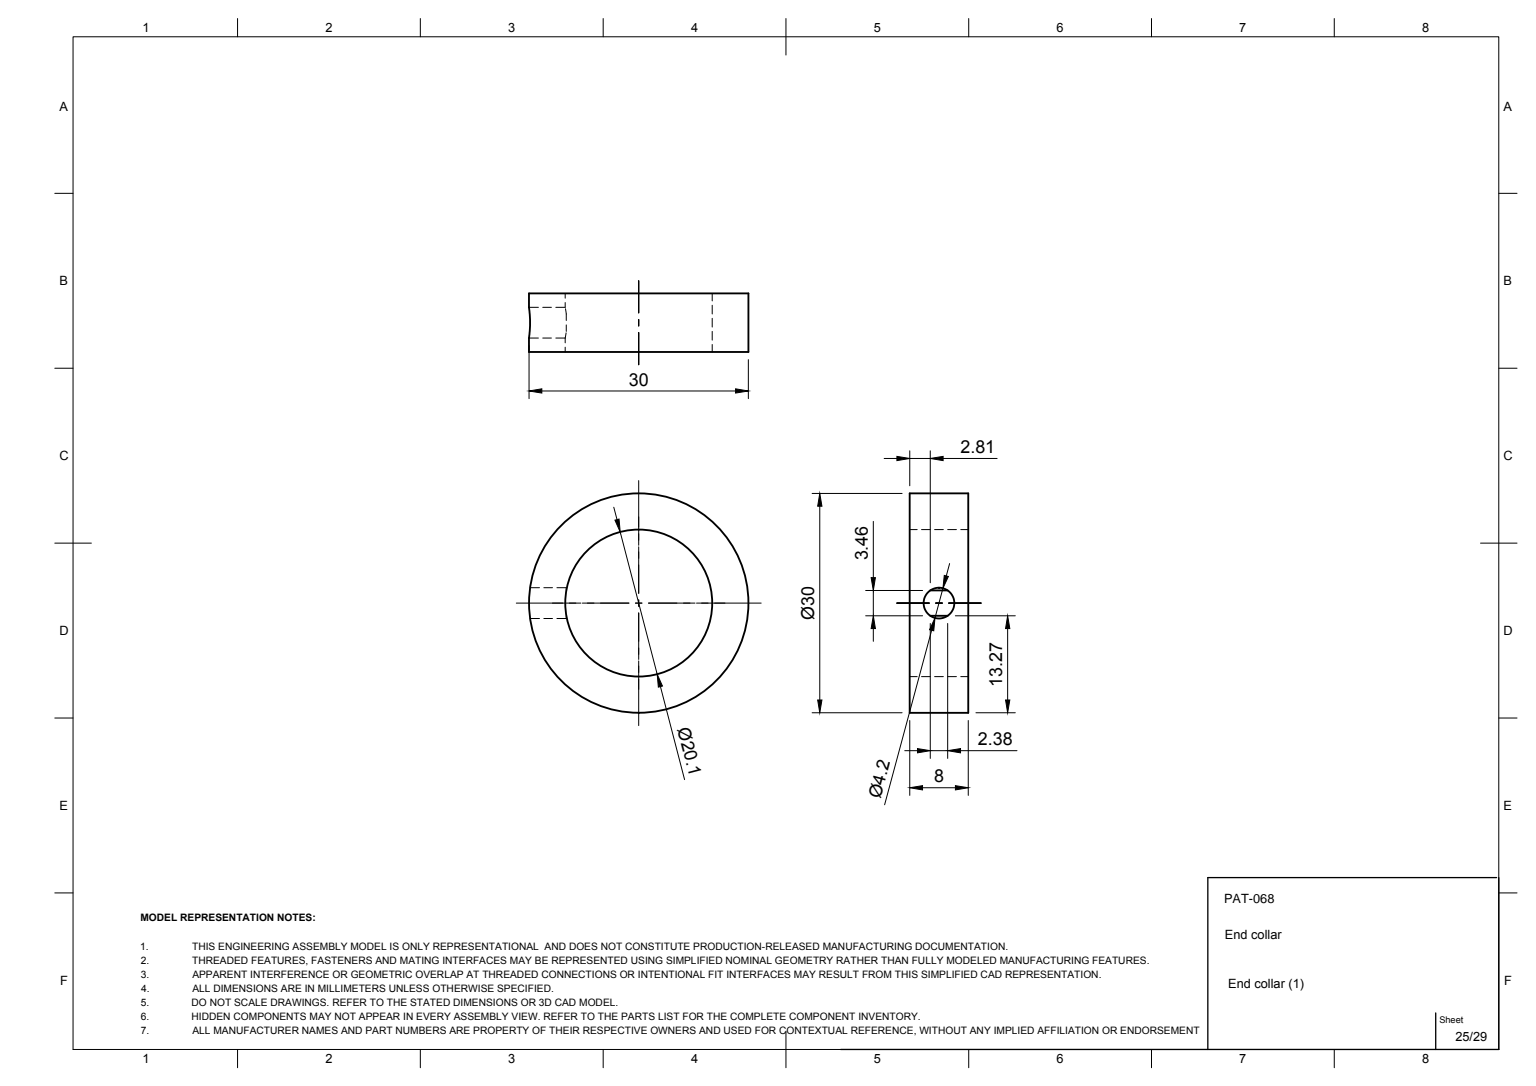
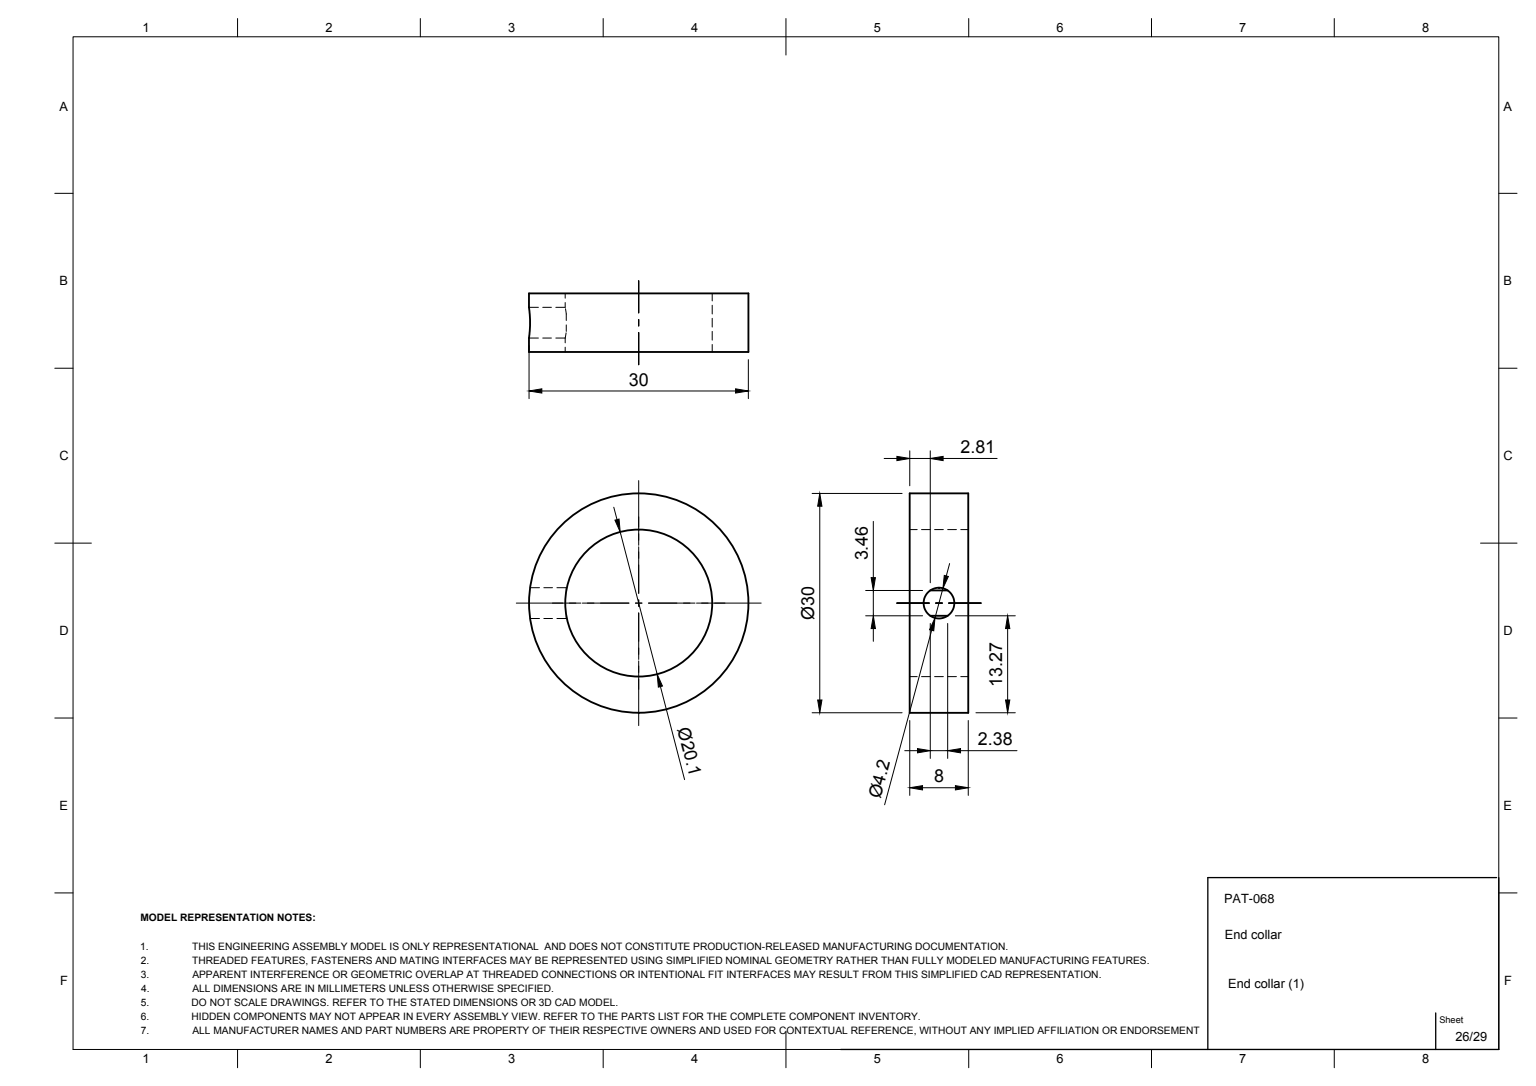
ISO-10303-21;
HEADER;
/* Generated by software containing ST-Developer
 * from STEP Tools, Inc. (www.steptools.com) 
 */

FILE_DESCRIPTION(
/* description */ ('Line shaft on three pillow blocks'),
/* implementation_level */ '2;1');

FILE_NAME(
/* name */ 'End collar.step',
/* time_stamp */ '2026-10-27T10:49:19-07:00',
/* author */ (''),
/* organization */ (''),
/* preprocessor_version */ 'ST-DEVELOPER v20.2',
/* originating_system */ 'Autodesk Translation Framework v15.17.0.0',
/* authorisation */ '');

FILE_SCHEMA (('AUTOMOTIVE_DESIGN { 1 0 10303 214 3 1 1 }'));
ENDSEC;

DATA;
#10=MECHANICAL_DESIGN_GEOMETRIC_PRESENTATION_REPRESENTATION('',(#359),#8377);
#255=B_SPLINE_CURVE_WITH_KNOTS('',3,(#7910,#7911,#7912,#7913,#7914,#7915,
#7916,#7917,#7918,#7919,#7920,#7921,#7922,#7923),.UNSPECIFIED.,.F.,.F.,
(4,2,2,2,2,2,4),(0.75600573798702,0.793568827564647,0.872922520054201,0.952276212543756,
1.03162990503331,1.11098359752287,1.14854668710049),.UNSPECIFIED.);
#256=B_SPLINE_CURVE_WITH_KNOTS('',3,(#7929,#7930,#7931,#7932,#7933,#7934,
#7935,#7936,#7937,#7938,#7939,#7940,#7941,#7942,#7943,#7944,#7945,#7946),
 .UNSPECIFIED.,.F.,.F.,(4,2,2,2,2,2,2,2,4),(0.,0.079216580773363,0.158433161546726,
0.23764869707457,0.316864232602414,0.396079768130259,0.475295303658103,
0.554511884431466,0.633728465204829),.UNSPECIFIED.);
#257=B_SPLINE_CURVE_WITH_KNOTS('',3,(#7947,#7948,#7949,#7950,#7951,#7952,
#7953,#7954,#7955,#7956,#7957,#7958,#7959,#7960,#7961,#7962,#7963,#7964),
 .UNSPECIFIED.,.F.,.F.,(4,2,2,2,2,2,2,2,4),(0.633728465204829,0.712945045978192,
0.792161626751555,0.871377162279399,0.950592697807244,1.02980823333509,
1.10902376886293,1.18824034963629,1.26745693040966),.UNSPECIFIED.);
#258=B_SPLINE_CURVE_WITH_KNOTS('',3,(#7967,#7968,#7969,#7970,#7971,#7972,
#7973,#7974,#7975,#7976,#7977,#7978,#7979,#7980),.UNSPECIFIED.,.F.,.F.,
(4,2,2,2,2,2,4),(0.121154929624515,0.158718019202143,0.238071711691697,
0.317425404181252,0.396779096670807,0.476132789160362,0.513695878737989),
 .UNSPECIFIED.);
#304=SHAPE_REPRESENTATION_RELATIONSHIP('SRR','None',#8521,#331);
#331=ADVANCED_BREP_SHAPE_REPRESENTATION('',(#385),#8370);
#359=STYLED_ITEM('',(#8704),#385);
#385=MANIFOLD_SOLID_BREP('Body1',#4347);
#474=FACE_BOUND('',#1184,.T.);
#475=FACE_BOUND('',#1186,.T.);
#476=FACE_BOUND('',#1188,.T.);
#477=FACE_BOUND('',#1190,.T.);
#612=PLANE('',#5030);
#613=PLANE('',#5035);
#614=PLANE('',#5042);
#615=PLANE('',#5043);
#845=FACE_OUTER_BOUND('',#1180,.T.);
#846=FACE_OUTER_BOUND('',#1181,.T.);
#847=FACE_OUTER_BOUND('',#1182,.T.);
#848=FACE_OUTER_BOUND('',#1183,.T.);
#849=FACE_OUTER_BOUND('',#1185,.T.);
#850=FACE_OUTER_BOUND('',#1187,.T.);
#851=FACE_OUTER_BOUND('',#1189,.T.);
#1180=EDGE_LOOP('',(#3751,#3752));
#1181=EDGE_LOOP('',(#3753,#3754,#3755,#3756,#3757,#3758,#3759,#3760,#3761));
#1182=EDGE_LOOP('',(#3762,#3763,#3764));
#1183=EDGE_LOOP('',(#3765,#3766,#3767,#3768));
#1184=EDGE_LOOP('',(#3769,#3770,#3771,#3772));
#1185=EDGE_LOOP('',(#3773,#3774,#3775,#3776));
#1186=EDGE_LOOP('',(#3777,#3778));
#1187=EDGE_LOOP('',(#3779));
#1188=EDGE_LOOP('',(#3780));
#1189=EDGE_LOOP('',(#3781));
#1190=EDGE_LOOP('',(#3782));
#1499=LINE('',#7906,#1826);
#1500=LINE('',#7927,#1827);
#1501=LINE('',#7982,#1828);
#1502=LINE('',#7987,#1829);
#1503=LINE('',#7993,#1830);
#1826=VECTOR('',#6148,1.);
#1827=VECTOR('',#6155,0.21);
#1828=VECTOR('',#6160,1.);
#1829=VECTOR('',#6165,1.005);
#1830=VECTOR('',#6172,1.5);
#2034=CIRCLE('',#5031,0.21);
#2035=CIRCLE('',#5033,0.21);
#2036=CIRCLE('',#5034,0.21);
#2037=CIRCLE('',#5037,1.005);
#2038=CIRCLE('',#5038,1.005);
#2039=CIRCLE('',#5040,1.5);
#2040=CIRCLE('',#5041,1.5);
#2341=VERTEX_POINT('',#7904);
#2342=VERTEX_POINT('',#7905);
#2343=VERTEX_POINT('',#7909);
#2344=VERTEX_POINT('',#7924);
#2345=VERTEX_POINT('',#7926);
#2346=VERTEX_POINT('',#7928);
#2347=VERTEX_POINT('',#7965);
#2348=VERTEX_POINT('',#7984);
#2349=VERTEX_POINT('',#7986);
#2350=VERTEX_POINT('',#7990);
#2351=VERTEX_POINT('',#7992);
#2824=EDGE_CURVE('',#2341,#2342,#1499,.T.);
#2825=EDGE_CURVE('',#2341,#2342,#2034,.T.);
#2826=EDGE_CURVE('',#2343,#2341,#255,.T.);
#2827=EDGE_CURVE('',#2344,#2343,#2035,.T.);
#2828=EDGE_CURVE('',#2344,#2345,#1500,.T.);
#2829=EDGE_CURVE('',#2346,#2345,#256,.T.);
#2830=EDGE_CURVE('',#2345,#2346,#257,.T.);
#2831=EDGE_CURVE('',#2347,#2344,#2036,.T.);
#2832=EDGE_CURVE('',#2342,#2347,#258,.T.);
#2833=EDGE_CURVE('',#2347,#2343,#1501,.T.);
#2834=EDGE_CURVE('',#2348,#2348,#2037,.T.);
#2835=EDGE_CURVE('',#2348,#2349,#1502,.T.);
#2836=EDGE_CURVE('',#2349,#2349,#2038,.T.);
#2837=EDGE_CURVE('',#2350,#2350,#2039,.T.);
#2838=EDGE_CURVE('',#2350,#2351,#1503,.T.);
#2839=EDGE_CURVE('',#2351,#2351,#2040,.T.);
#3751=ORIENTED_EDGE('',*,*,#2824,.F.);
#3752=ORIENTED_EDGE('',*,*,#2825,.T.);
#3753=ORIENTED_EDGE('',*,*,#2826,.F.);
#3754=ORIENTED_EDGE('',*,*,#2827,.F.);
#3755=ORIENTED_EDGE('',*,*,#2828,.T.);
#3756=ORIENTED_EDGE('',*,*,#2829,.F.);
#3757=ORIENTED_EDGE('',*,*,#2830,.F.);
#3758=ORIENTED_EDGE('',*,*,#2828,.F.);
#3759=ORIENTED_EDGE('',*,*,#2831,.F.);
#3760=ORIENTED_EDGE('',*,*,#2832,.F.);
#3761=ORIENTED_EDGE('',*,*,#2825,.F.);
#3762=ORIENTED_EDGE('',*,*,#2833,.F.);
#3763=ORIENTED_EDGE('',*,*,#2831,.T.);
#3764=ORIENTED_EDGE('',*,*,#2827,.T.);
#3765=ORIENTED_EDGE('',*,*,#2834,.F.);
#3766=ORIENTED_EDGE('',*,*,#2835,.T.);
#3767=ORIENTED_EDGE('',*,*,#2836,.T.);
#3768=ORIENTED_EDGE('',*,*,#2835,.F.);
#3769=ORIENTED_EDGE('',*,*,#2832,.T.);
#3770=ORIENTED_EDGE('',*,*,#2833,.T.);
#3771=ORIENTED_EDGE('',*,*,#2826,.T.);
#3772=ORIENTED_EDGE('',*,*,#2824,.T.);
#3773=ORIENTED_EDGE('',*,*,#2837,.F.);
#3774=ORIENTED_EDGE('',*,*,#2838,.T.);
#3775=ORIENTED_EDGE('',*,*,#2839,.T.);
#3776=ORIENTED_EDGE('',*,*,#2838,.F.);
#3777=ORIENTED_EDGE('',*,*,#2829,.T.);
#3778=ORIENTED_EDGE('',*,*,#2830,.T.);
#3779=ORIENTED_EDGE('',*,*,#2837,.T.);
#3780=ORIENTED_EDGE('',*,*,#2834,.T.);
#3781=ORIENTED_EDGE('',*,*,#2839,.F.);
#3782=ORIENTED_EDGE('',*,*,#2836,.F.);
#4059=CYLINDRICAL_SURFACE('',#5032,0.21);
#4060=CYLINDRICAL_SURFACE('',#5036,1.005);
#4061=CYLINDRICAL_SURFACE('',#5039,1.5);
#4263=ADVANCED_FACE('',(#845),#612,.T.);
#4264=ADVANCED_FACE('',(#846),#4059,.F.);
#4265=ADVANCED_FACE('',(#847),#613,.T.);
#4266=ADVANCED_FACE('',(#848,#474),#4060,.F.);
#4267=ADVANCED_FACE('',(#849,#475),#4061,.T.);
#4268=ADVANCED_FACE('',(#850,#476),#614,.T.);
#4269=ADVANCED_FACE('',(#851,#477),#615,.F.);
#4347=CLOSED_SHELL('',(#4263,#4264,#4265,#4266,#4267,#4268,#4269));
#5029=AXIS2_PLACEMENT_3D('',#7902,#6144,#6145);
#5030=AXIS2_PLACEMENT_3D('',#7903,#6146,#6147);
#5031=AXIS2_PLACEMENT_3D('',#7907,#6149,#6150);
#5032=AXIS2_PLACEMENT_3D('',#7908,#6151,#6152);
#5033=AXIS2_PLACEMENT_3D('',#7925,#6153,#6154);
#5034=AXIS2_PLACEMENT_3D('',#7966,#6156,#6157);
#5035=AXIS2_PLACEMENT_3D('',#7981,#6158,#6159);
#5036=AXIS2_PLACEMENT_3D('',#7983,#6161,#6162);
#5037=AXIS2_PLACEMENT_3D('',#7985,#6163,#6164);
#5038=AXIS2_PLACEMENT_3D('',#7988,#6166,#6167);
#5039=AXIS2_PLACEMENT_3D('',#7989,#6168,#6169);
#5040=AXIS2_PLACEMENT_3D('',#7991,#6170,#6171);
#5041=AXIS2_PLACEMENT_3D('',#7994,#6173,#6174);
#5042=AXIS2_PLACEMENT_3D('',#7995,#6175,#6176);
#5043=AXIS2_PLACEMENT_3D('',#7996,#6177,#6178);
#6144=DIRECTION('axis',(0.,0.,1.));
#6145=DIRECTION('refdir',(1.,0.,0.));
#6146=DIRECTION('center_axis',(0.,0.,1.));
#6147=DIRECTION('ref_axis',(1.,0.,0.));
#6148=DIRECTION('',(0.,1.,0.));
#6149=DIRECTION('center_axis',(0.,0.,1.));
#6150=DIRECTION('ref_axis',(1.,0.,0.));
#6151=DIRECTION('center_axis',(0.,0.,1.));
#6152=DIRECTION('ref_axis',(1.,0.,0.));
#6153=DIRECTION('center_axis',(0.,0.,1.));
#6154=DIRECTION('ref_axis',(1.,0.,0.));
#6155=DIRECTION('',(0.,0.,1.));
#6156=DIRECTION('center_axis',(0.,0.,1.));
#6157=DIRECTION('ref_axis',(1.,0.,0.));
#6158=DIRECTION('center_axis',(0.,0.,1.));
#6159=DIRECTION('ref_axis',(1.,0.,0.));
#6160=DIRECTION('',(0.,-1.,0.));
#6161=DIRECTION('center_axis',(0.,1.,0.));
#6162=DIRECTION('ref_axis',(1.,0.,0.));
#6163=DIRECTION('center_axis',(0.,-1.,0.));
#6164=DIRECTION('ref_axis',(1.,0.,0.));
#6165=DIRECTION('',(0.,-1.,0.));
#6166=DIRECTION('center_axis',(0.,-1.,0.));
#6167=DIRECTION('ref_axis',(1.,0.,0.));
#6168=DIRECTION('center_axis',(0.,1.,0.));
#6169=DIRECTION('ref_axis',(1.,0.,0.));
#6170=DIRECTION('center_axis',(0.,1.,0.));
#6171=DIRECTION('ref_axis',(1.,0.,0.));
#6172=DIRECTION('',(0.,-1.,0.));
#6173=DIRECTION('center_axis',(0.,1.,0.));
#6174=DIRECTION('ref_axis',(1.,0.,0.));
#6175=DIRECTION('center_axis',(0.,1.,0.));
#6176=DIRECTION('ref_axis',(1.,0.,0.));
#6177=DIRECTION('center_axis',(0.,1.,0.));
#6178=DIRECTION('ref_axis',(1.,0.,0.));
#7902=CARTESIAN_POINT('',(0.,0.,0.));
#7903=CARTESIAN_POINT('Origin',(0.,-1.25,5.52));
#7904=CARTESIAN_POINT('',(0.172988438920056,-1.36905880899792,5.52));
#7905=CARTESIAN_POINT('',(0.172988438920056,-1.13094119100209,5.52));
#7906=CARTESIAN_POINT('',(0.172988438920056,-1.65,5.52));
#7907=CARTESIAN_POINT('Origin',(0.,-1.25,5.52));
#7908=CARTESIAN_POINT('Origin',(0.,-1.25,5.52));
#7909=CARTESIAN_POINT('',(-0.172988438920056,-1.36905880899792,5.52));
#7910=CARTESIAN_POINT('Ctrl Pts',(-0.172988438920056,-1.36905880899792,
5.52));
#7911=CARTESIAN_POINT('Ctrl Pts',(-0.165594865311314,-1.37980142239529,
5.52129192197638));
#7912=CARTESIAN_POINT('Ctrl Pts',(-0.157297138725606,-1.38968770937274,
5.52265394943905));
#7913=CARTESIAN_POINT('Ctrl Pts',(-0.129892073845076,-1.41709277425327,
5.5267480843909));
#7914=CARTESIAN_POINT('Ctrl Pts',(-0.106330167759284,-1.43324205633295,
5.52969589327638));
#7915=CARTESIAN_POINT('Ctrl Pts',(-0.0546129046324105,-1.45469779396491,
5.53385029472357));
#7916=CARTESIAN_POINT('Ctrl Pts',(-0.0264512308298517,-1.46,5.535));
#7917=CARTESIAN_POINT('Ctrl Pts',(0.0264512308298516,-1.46,5.535));
#7918=CARTESIAN_POINT('Ctrl Pts',(0.0546129046324104,-1.45469779396491,
5.53385029472357));
#7919=CARTESIAN_POINT('Ctrl Pts',(0.106330167759284,-1.43324205633295,5.52969589327638));
#7920=CARTESIAN_POINT('Ctrl Pts',(0.129892073845076,-1.41709277425327,5.5267480843909));
#7921=CARTESIAN_POINT('Ctrl Pts',(0.157297138725606,-1.38968770937274,5.52265394943905));
#7922=CARTESIAN_POINT('Ctrl Pts',(0.165594865311314,-1.37980142239529,5.52129192197638));
#7923=CARTESIAN_POINT('Ctrl Pts',(0.172988438920056,-1.36905880899792,5.52));
#7924=CARTESIAN_POINT('',(-0.21,-1.25,5.52));
#7925=CARTESIAN_POINT('Origin',(0.,-1.25,5.52));
#7926=CARTESIAN_POINT('',(-0.21,-1.25,6.01522725533839));
#7927=CARTESIAN_POINT('',(-0.21,-1.25,5.52));
#7928=CARTESIAN_POINT('',(0.21,-1.25,6.01522725533839));
#7929=CARTESIAN_POINT('Ctrl Pts',(0.21,-1.25,6.01522725533839));
#7930=CARTESIAN_POINT('Ctrl Pts',(0.21,-1.27640552692445,6.01522725533839));
#7931=CARTESIAN_POINT('Ctrl Pts',(0.204715737269596,-1.30454707409071,6.01600415954412));
#7932=CARTESIAN_POINT('Ctrl Pts',(0.183273763036331,-1.35627626890513,6.01880073282317));
#7933=CARTESIAN_POINT('Ctrl Pts',(0.167117923970394,-1.37986692412796,6.02077897157582));
#7934=CARTESIAN_POINT('Ctrl Pts',(0.129867169887369,-1.41711767821098,6.02448481141327));
#7935=CARTESIAN_POINT('Ctrl Pts',(0.106276408305765,-1.43327371000135,6.02645455657129));
#7936=CARTESIAN_POINT('Ctrl Pts',(0.0545468514059002,-1.45471582482622,
6.02923165515645));
#7937=CARTESIAN_POINT('Ctrl Pts',(0.0264051785092814,-1.46,6.03));
#7938=CARTESIAN_POINT('Ctrl Pts',(-0.0264051785092814,-1.46,6.03));
#7939=CARTESIAN_POINT('Ctrl Pts',(-0.0545468514059001,-1.45471582482622,
6.02923165515645));
#7940=CARTESIAN_POINT('Ctrl Pts',(-0.106276408305765,-1.43327371000135,
6.02645455657129));
#7941=CARTESIAN_POINT('Ctrl Pts',(-0.129867169887369,-1.41711767821098,
6.02448481141327));
#7942=CARTESIAN_POINT('Ctrl Pts',(-0.167117923970394,-1.37986692412796,
6.02077897157582));
#7943=CARTESIAN_POINT('Ctrl Pts',(-0.183273763036331,-1.35627626890513,
6.01880073282317));
#7944=CARTESIAN_POINT('Ctrl Pts',(-0.204715737269596,-1.30454707409071,
6.01600415954412));
#7945=CARTESIAN_POINT('Ctrl Pts',(-0.21,-1.27640552692445,6.01522725533839));
#7946=CARTESIAN_POINT('Ctrl Pts',(-0.21,-1.25,6.01522725533839));
#7947=CARTESIAN_POINT('Ctrl Pts',(-0.21,-1.25,6.01522725533839));
#7948=CARTESIAN_POINT('Ctrl Pts',(-0.21,-1.22359447307555,6.01522725533839));
#7949=CARTESIAN_POINT('Ctrl Pts',(-0.204715737269596,-1.19545292590929,
6.01600415954412));
#7950=CARTESIAN_POINT('Ctrl Pts',(-0.183273763036331,-1.14372373109487,
6.01880073282317));
#7951=CARTESIAN_POINT('Ctrl Pts',(-0.167117923970394,-1.12013307587204,
6.02077897157582));
#7952=CARTESIAN_POINT('Ctrl Pts',(-0.129867169887369,-1.08288232178902,
6.02448481141327));
#7953=CARTESIAN_POINT('Ctrl Pts',(-0.106276408305765,-1.06672628999865,
6.02645455657129));
#7954=CARTESIAN_POINT('Ctrl Pts',(-0.0545468514059002,-1.04528417517378,
6.02923165515645));
#7955=CARTESIAN_POINT('Ctrl Pts',(-0.0264051785092814,-1.04,6.03));
#7956=CARTESIAN_POINT('Ctrl Pts',(0.0264051785092814,-1.04,6.03));
#7957=CARTESIAN_POINT('Ctrl Pts',(0.0545468514059001,-1.04528417517378,
6.02923165515645));
#7958=CARTESIAN_POINT('Ctrl Pts',(0.106276408305765,-1.06672628999865,6.02645455657129));
#7959=CARTESIAN_POINT('Ctrl Pts',(0.129867169887369,-1.08288232178902,6.02448481141327));
#7960=CARTESIAN_POINT('Ctrl Pts',(0.167117923970394,-1.12013307587204,6.02077897157582));
#7961=CARTESIAN_POINT('Ctrl Pts',(0.183273763036331,-1.14372373109487,6.01880073282317));
#7962=CARTESIAN_POINT('Ctrl Pts',(0.204715737269596,-1.19545292590929,6.01600415954412));
#7963=CARTESIAN_POINT('Ctrl Pts',(0.21,-1.22359447307555,6.01522725533839));
#7964=CARTESIAN_POINT('Ctrl Pts',(0.21,-1.25,6.01522725533839));
#7965=CARTESIAN_POINT('',(-0.172988438920056,-1.13094119100209,5.52));
#7966=CARTESIAN_POINT('Origin',(0.,-1.25,5.52));
#7967=CARTESIAN_POINT('Ctrl Pts',(0.172988438920056,-1.13094119100209,5.52));
#7968=CARTESIAN_POINT('Ctrl Pts',(0.165594865311315,-1.12019857760471,5.52129192197638));
#7969=CARTESIAN_POINT('Ctrl Pts',(0.157297138725606,-1.11031229062726,5.52265394943905));
#7970=CARTESIAN_POINT('Ctrl Pts',(0.129892073845076,-1.08290722574673,5.5267480843909));
#7971=CARTESIAN_POINT('Ctrl Pts',(0.106330167759284,-1.06675794366705,5.52969589327638));
#7972=CARTESIAN_POINT('Ctrl Pts',(0.0546129046324104,-1.04530220603509,
5.53385029472357));
#7973=CARTESIAN_POINT('Ctrl Pts',(0.0264512308298516,-1.04,5.535));
#7974=CARTESIAN_POINT('Ctrl Pts',(-0.0264512308298516,-1.04,5.535));
#7975=CARTESIAN_POINT('Ctrl Pts',(-0.0546129046324104,-1.04530220603509,
5.53385029472357));
#7976=CARTESIAN_POINT('Ctrl Pts',(-0.106330167759284,-1.06675794366705,
5.52969589327638));
#7977=CARTESIAN_POINT('Ctrl Pts',(-0.129892073845076,-1.08290722574673,
5.5267480843909));
#7978=CARTESIAN_POINT('Ctrl Pts',(-0.157297138725606,-1.11031229062726,
5.52265394943905));
#7979=CARTESIAN_POINT('Ctrl Pts',(-0.165594865311315,-1.12019857760471,
5.52129192197638));
#7980=CARTESIAN_POINT('Ctrl Pts',(-0.172988438920056,-1.13094119100209,
5.52));
#7981=CARTESIAN_POINT('Origin',(0.,-1.25,5.52));
#7982=CARTESIAN_POINT('',(-0.172988438920056,-1.65,5.52));
#7983=CARTESIAN_POINT('Origin',(0.,-1.65,4.53));
#7984=CARTESIAN_POINT('',(-1.005,-0.85,4.53));
#7985=CARTESIAN_POINT('Origin',(0.,-0.85,4.53));
#7986=CARTESIAN_POINT('',(-1.005,-1.65,4.53));
#7987=CARTESIAN_POINT('',(-1.005,-1.65,4.53));
#7988=CARTESIAN_POINT('Origin',(0.,-1.65,4.53));
#7989=CARTESIAN_POINT('Origin',(0.,-1.65,4.53));
#7990=CARTESIAN_POINT('',(-1.5,-0.85,4.53));
#7991=CARTESIAN_POINT('Origin',(0.,-0.85,4.53));
#7992=CARTESIAN_POINT('',(-1.5,-1.65,4.53));
#7993=CARTESIAN_POINT('',(-1.5,-1.65,4.53));
#7994=CARTESIAN_POINT('Origin',(0.,-1.65,4.53));
#7995=CARTESIAN_POINT('Origin',(0.,-0.85,4.53));
#7996=CARTESIAN_POINT('Origin',(0.,-1.65,4.53));
#8338=UNCERTAINTY_MEASURE_WITH_UNIT(LENGTH_MEASURE(0.001),#8378,
'DISTANCE_ACCURACY_VALUE',
'Maximum model space distance between geometric entities at asserted c
onnectivities');
#8345=UNCERTAINTY_MEASURE_WITH_UNIT(LENGTH_MEASURE(0.001),#8378,
'DISTANCE_ACCURACY_VALUE',
'Maximum model space distance between geometric entities at asserted c
onnectivities');
#8370=(
GEOMETRIC_REPRESENTATION_CONTEXT(3)
GLOBAL_UNCERTAINTY_ASSIGNED_CONTEXT((#8338))
GLOBAL_UNIT_ASSIGNED_CONTEXT((#8378,#8380,#8381))
REPRESENTATION_CONTEXT('','3D')
);
#8377=(
GEOMETRIC_REPRESENTATION_CONTEXT(3)
GLOBAL_UNCERTAINTY_ASSIGNED_CONTEXT((#8345))
GLOBAL_UNIT_ASSIGNED_CONTEXT((#8378,#8380,#8381))
REPRESENTATION_CONTEXT('','3D')
);
#8378=(
LENGTH_UNIT()
NAMED_UNIT(*)
SI_UNIT(.CENTI.,.METRE.)
);
#8380=(
NAMED_UNIT(*)
PLANE_ANGLE_UNIT()
SI_UNIT($,.RADIAN.)
);
#8381=(
NAMED_UNIT(*)
SI_UNIT($,.STERADIAN.)
SOLID_ANGLE_UNIT()
);
#8406=SHAPE_DEFINITION_REPRESENTATION(#8473,#8521);
#8473=PRODUCT_DEFINITION_SHAPE('',$,#8553);
#8521=SHAPE_REPRESENTATION('',(#5029),#8370);
#8528=PRODUCT_DEFINITION_CONTEXT('part definition',#8623,'design');
#8553=PRODUCT_DEFINITION('End collar','End collar',#8584,#8528);
#8584=PRODUCT_DEFINITION_FORMATION('',$,#8649);
#8623=APPLICATION_CONTEXT(
'Core Data for Automotive Mechanical Design Process');
#8624=PRODUCT_CONTEXT('part definition',#8623,'mechanical');
#8649=PRODUCT('End collar','End collar','End collar',(#8624));
#8698=COLOUR_RGB('Light Blue',0.38,0.62,0.78);
#8699=FILL_AREA_STYLE_COLOUR('',#8698);
#8700=FILL_AREA_STYLE('',(#8699));
#8701=SURFACE_STYLE_FILL_AREA(#8700);
#8702=SURFACE_SIDE_STYLE('',(#8701));
#8703=SURFACE_STYLE_USAGE(.BOTH.,#8702);
#8704=PRESENTATION_STYLE_ASSIGNMENT((#8703));
ENDSEC;
END-ISO-10303-21;
